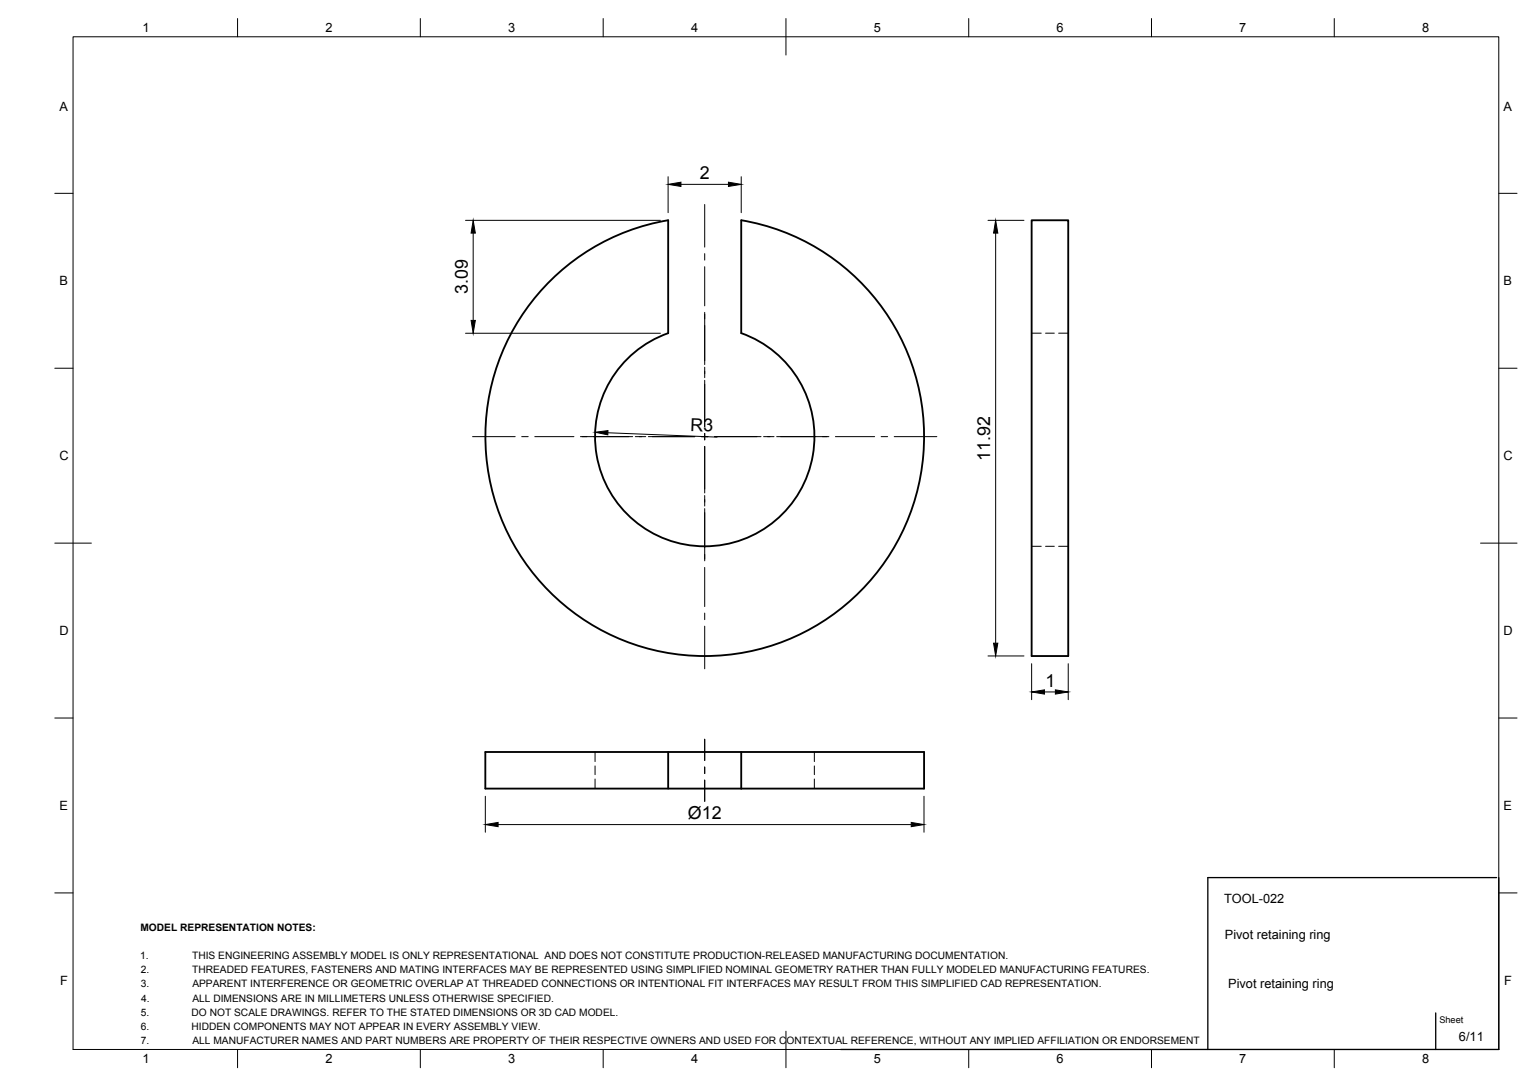
ISO-10303-21;
HEADER;
/* Generated by software containing ST-Developer
 * from STEP Tools, Inc. (www.steptools.com) 
 */

FILE_DESCRIPTION(
/* description */ (''),
/* implementation_level */ '2;1');

FILE_NAME(
/* name */ 'Pivot retaining ring.step',
/* time_stamp */ '2026-11-10T08:27:36-08:00',
/* author */ (''),
/* organization */ (''),
/* preprocessor_version */ 'ST-DEVELOPER v20.2',
/* originating_system */ 'Autodesk Translation Framework v15.17.0.0',
/* authorisation */ '');

FILE_SCHEMA (('AUTOMOTIVE_DESIGN { 1 0 10303 214 3 1 1 }'));
ENDSEC;

DATA;
#10=MECHANICAL_DESIGN_GEOMETRIC_PRESENTATION_REPRESENTATION('',(#569),#19090);
#549=SHAPE_REPRESENTATION_RELATIONSHIP('SRR','None',#19139,#559);
#559=ADVANCED_BREP_SHAPE_REPRESENTATION('',(#579),#19082);
#569=STYLED_ITEM('',(#19202),#579);
#579=MANIFOLD_SOLID_BREP('Body1',#6823);
#695=PLANE('',#7030);
#696=PLANE('',#7031);
#697=PLANE('',#7032);
#698=PLANE('',#7039);
#869=FACE_OUTER_BOUND('',#1272,.T.);
#870=FACE_OUTER_BOUND('',#1273,.T.);
#871=FACE_OUTER_BOUND('',#1274,.T.);
#872=FACE_OUTER_BOUND('',#1275,.T.);
#873=FACE_OUTER_BOUND('',#1276,.T.);
#874=FACE_OUTER_BOUND('',#1277,.T.);
#1272=EDGE_LOOP('',(#4609,#4610,#4611,#4612));
#1273=EDGE_LOOP('',(#4613,#4614,#4615,#4616));
#1274=EDGE_LOOP('',(#4617,#4618,#4619,#4620));
#1275=EDGE_LOOP('',(#4621,#4622,#4623,#4624));
#1276=EDGE_LOOP('',(#4625,#4626,#4627,#4628));
#1277=EDGE_LOOP('',(#4629,#4630,#4631,#4632));
#1765=LINE('',#9169,#2214);
#1766=LINE('',#9171,#2215);
#1767=LINE('',#9173,#2216);
#1768=LINE('',#9174,#2217);
#1769=LINE('',#9178,#2218);
#1770=LINE('',#9180,#2219);
#1771=LINE('',#9182,#2220);
#1772=LINE('',#9183,#2221);
#2214=VECTOR('',#7726,1.);
#2215=VECTOR('',#7727,1.);
#2216=VECTOR('',#7728,1.);
#2217=VECTOR('',#7729,1.);
#2218=VECTOR('',#7732,1.);
#2219=VECTOR('',#7733,1.);
#2220=VECTOR('',#7734,1.);
#2221=VECTOR('',#7735,1.);
#2582=CIRCLE('',#7033,0.6);
#2583=CIRCLE('',#7034,0.3);
#2584=CIRCLE('',#7036,0.3);
#2585=CIRCLE('',#7038,0.6);
#2804=VERTEX_POINT('',#9167);
#2805=VERTEX_POINT('',#9168);
#2806=VERTEX_POINT('',#9170);
#2807=VERTEX_POINT('',#9172);
#2808=VERTEX_POINT('',#9176);
#2809=VERTEX_POINT('',#9177);
#2810=VERTEX_POINT('',#9179);
#2811=VERTEX_POINT('',#9181);
#3489=EDGE_CURVE('',#2804,#2805,#1765,.T.);
#3490=EDGE_CURVE('',#2806,#2804,#1766,.T.);
#3491=EDGE_CURVE('',#2807,#2806,#1767,.T.);
#3492=EDGE_CURVE('',#2805,#2807,#1768,.T.);
#3493=EDGE_CURVE('',#2808,#2809,#1769,.T.);
#3494=EDGE_CURVE('',#2810,#2808,#1770,.T.);
#3495=EDGE_CURVE('',#2811,#2810,#1771,.T.);
#3496=EDGE_CURVE('',#2809,#2811,#1772,.T.);
#3497=EDGE_CURVE('',#2806,#2811,#2582,.T.);
#3498=EDGE_CURVE('',#2809,#2804,#2583,.T.);
#3499=EDGE_CURVE('',#2808,#2805,#2584,.T.);
#3500=EDGE_CURVE('',#2807,#2810,#2585,.T.);
#4609=ORIENTED_EDGE('',*,*,#3489,.F.);
#4610=ORIENTED_EDGE('',*,*,#3490,.F.);
#4611=ORIENTED_EDGE('',*,*,#3491,.F.);
#4612=ORIENTED_EDGE('',*,*,#3492,.F.);
#4613=ORIENTED_EDGE('',*,*,#3493,.F.);
#4614=ORIENTED_EDGE('',*,*,#3494,.F.);
#4615=ORIENTED_EDGE('',*,*,#3495,.F.);
#4616=ORIENTED_EDGE('',*,*,#3496,.F.);
#4617=ORIENTED_EDGE('',*,*,#3496,.T.);
#4618=ORIENTED_EDGE('',*,*,#3497,.F.);
#4619=ORIENTED_EDGE('',*,*,#3490,.T.);
#4620=ORIENTED_EDGE('',*,*,#3498,.F.);
#4621=ORIENTED_EDGE('',*,*,#3493,.T.);
#4622=ORIENTED_EDGE('',*,*,#3498,.T.);
#4623=ORIENTED_EDGE('',*,*,#3489,.T.);
#4624=ORIENTED_EDGE('',*,*,#3499,.F.);
#4625=ORIENTED_EDGE('',*,*,#3495,.T.);
#4626=ORIENTED_EDGE('',*,*,#3500,.F.);
#4627=ORIENTED_EDGE('',*,*,#3491,.T.);
#4628=ORIENTED_EDGE('',*,*,#3497,.T.);
#4629=ORIENTED_EDGE('',*,*,#3494,.T.);
#4630=ORIENTED_EDGE('',*,*,#3499,.T.);
#4631=ORIENTED_EDGE('',*,*,#3492,.T.);
#4632=ORIENTED_EDGE('',*,*,#3500,.T.);
#6315=CYLINDRICAL_SURFACE('',#7035,0.3);
#6316=CYLINDRICAL_SURFACE('',#7037,0.6);
#6488=ADVANCED_FACE('',(#869),#695,.F.);
#6489=ADVANCED_FACE('',(#870),#696,.F.);
#6490=ADVANCED_FACE('',(#871),#697,.F.);
#6491=ADVANCED_FACE('',(#872),#6315,.F.);
#6492=ADVANCED_FACE('',(#873),#6316,.T.);
#6493=ADVANCED_FACE('',(#874),#698,.T.);
#6823=CLOSED_SHELL('',(#6488,#6489,#6490,#6491,#6492,#6493));
#7029=AXIS2_PLACEMENT_3D('',#9165,#7722,#7723);
#7030=AXIS2_PLACEMENT_3D('',#9166,#7724,#7725);
#7031=AXIS2_PLACEMENT_3D('',#9175,#7730,#7731);
#7032=AXIS2_PLACEMENT_3D('',#9184,#7736,#7737);
#7033=AXIS2_PLACEMENT_3D('',#9185,#7738,#7739);
#7034=AXIS2_PLACEMENT_3D('',#9186,#7740,#7741);
#7035=AXIS2_PLACEMENT_3D('',#9187,#7742,#7743);
#7036=AXIS2_PLACEMENT_3D('',#9188,#7744,#7745);
#7037=AXIS2_PLACEMENT_3D('',#9189,#7746,#7747);
#7038=AXIS2_PLACEMENT_3D('',#9190,#7748,#7749);
#7039=AXIS2_PLACEMENT_3D('',#9191,#7750,#7751);
#7722=DIRECTION('axis',(0.,0.,1.));
#7723=DIRECTION('refdir',(1.,0.,0.));
#7724=DIRECTION('center_axis',(-1.,0.,0.));
#7725=DIRECTION('ref_axis',(0.,1.,0.));
#7726=DIRECTION('',(0.,0.,1.));
#7727=DIRECTION('',(0.,-1.,0.));
#7728=DIRECTION('',(0.,0.,-1.));
#7729=DIRECTION('',(0.,1.,0.));
#7730=DIRECTION('center_axis',(1.,0.,0.));
#7731=DIRECTION('ref_axis',(0.,-1.,0.));
#7732=DIRECTION('',(0.,0.,-1.));
#7733=DIRECTION('',(0.,-1.,0.));
#7734=DIRECTION('',(0.,0.,1.));
#7735=DIRECTION('',(0.,1.,0.));
#7736=DIRECTION('center_axis',(0.,0.,1.));
#7737=DIRECTION('ref_axis',(1.,0.,0.));
#7738=DIRECTION('center_axis',(0.,0.,1.));
#7739=DIRECTION('ref_axis',(1.,0.,0.));
#7740=DIRECTION('center_axis',(0.,0.,-1.));
#7741=DIRECTION('ref_axis',(1.,0.,0.));
#7742=DIRECTION('center_axis',(0.,0.,1.));
#7743=DIRECTION('ref_axis',(6.12323399573677E-17,-1.,0.));
#7744=DIRECTION('center_axis',(0.,0.,-1.));
#7745=DIRECTION('ref_axis',(1.,0.,0.));
#7746=DIRECTION('center_axis',(0.,0.,1.));
#7747=DIRECTION('ref_axis',(6.12323399573677E-17,-1.,0.));
#7748=DIRECTION('center_axis',(0.,0.,1.));
#7749=DIRECTION('ref_axis',(1.,0.,0.));
#7750=DIRECTION('center_axis',(0.,0.,1.));
#7751=DIRECTION('ref_axis',(1.,0.,0.));
#9165=CARTESIAN_POINT('',(0.,0.,0.));
#9166=CARTESIAN_POINT('Origin',(-0.1,0.,0.1));
#9167=CARTESIAN_POINT('',(-0.1,0.282842712474619,0.));
#9168=CARTESIAN_POINT('',(-0.1,0.282842712474619,0.1));
#9169=CARTESIAN_POINT('',(-0.1,0.282842712474619,0.));
#9170=CARTESIAN_POINT('',(-0.1,0.591607978309962,0.));
#9171=CARTESIAN_POINT('',(-0.1,0.,0.));
#9172=CARTESIAN_POINT('',(-0.1,0.591607978309962,0.1));
#9173=CARTESIAN_POINT('',(-0.1,0.591607978309962,0.));
#9174=CARTESIAN_POINT('',(-0.1,0.,0.1));
#9175=CARTESIAN_POINT('Origin',(0.1,1.2,0.1));
#9176=CARTESIAN_POINT('',(0.1,0.282842712474619,0.1));
#9177=CARTESIAN_POINT('',(0.1,0.282842712474619,0.));
#9178=CARTESIAN_POINT('',(0.1,0.282842712474619,0.));
#9179=CARTESIAN_POINT('',(0.1,0.591607978309962,0.1));
#9180=CARTESIAN_POINT('',(0.1,0.6,0.1));
#9181=CARTESIAN_POINT('',(0.1,0.591607978309962,0.));
#9182=CARTESIAN_POINT('',(0.1,0.591607978309962,0.));
#9183=CARTESIAN_POINT('',(0.1,0.6,0.));
#9184=CARTESIAN_POINT('Origin',(0.,0.,0.));
#9185=CARTESIAN_POINT('Origin',(0.,0.,0.));
#9186=CARTESIAN_POINT('Origin',(0.,0.,0.));
#9187=CARTESIAN_POINT('Origin',(0.,0.,0.));
#9188=CARTESIAN_POINT('Origin',(0.,0.,0.1));
#9189=CARTESIAN_POINT('Origin',(0.,0.,0.));
#9190=CARTESIAN_POINT('Origin',(0.,0.,0.1));
#9191=CARTESIAN_POINT('Origin',(0.,0.,0.1));
#19069=UNCERTAINTY_MEASURE_WITH_UNIT(LENGTH_MEASURE(0.001),#19091,
'DISTANCE_ACCURACY_VALUE',
'Maximum model space distance between geometric entities at asserted c
onnectivities');
#19077=UNCERTAINTY_MEASURE_WITH_UNIT(LENGTH_MEASURE(0.001),#19091,
'DISTANCE_ACCURACY_VALUE',
'Maximum model space distance between geometric entities at asserted c
onnectivities');
#19082=(
GEOMETRIC_REPRESENTATION_CONTEXT(3)
GLOBAL_UNCERTAINTY_ASSIGNED_CONTEXT((#19069))
GLOBAL_UNIT_ASSIGNED_CONTEXT((#19091,#19093,#19094))
REPRESENTATION_CONTEXT('','3D')
);
#19090=(
GEOMETRIC_REPRESENTATION_CONTEXT(3)
GLOBAL_UNCERTAINTY_ASSIGNED_CONTEXT((#19077))
GLOBAL_UNIT_ASSIGNED_CONTEXT((#19091,#19093,#19094))
REPRESENTATION_CONTEXT('','3D')
);
#19091=(
LENGTH_UNIT()
NAMED_UNIT(*)
SI_UNIT(.CENTI.,.METRE.)
);
#19093=(
NAMED_UNIT(*)
PLANE_ANGLE_UNIT()
SI_UNIT($,.RADIAN.)
);
#19094=(
NAMED_UNIT(*)
SI_UNIT($,.STERADIAN.)
SOLID_ANGLE_UNIT()
);
#19099=SHAPE_DEFINITION_REPRESENTATION(#19111,#19139);
#19111=PRODUCT_DEFINITION_SHAPE('',$,#19152);
#19139=SHAPE_REPRESENTATION('',(#7029),#19082);
#19147=PRODUCT_DEFINITION_CONTEXT('part definition',#19185,'design');
#19152=PRODUCT_DEFINITION('Pivot retaining ring','Pivot retaining ring',
#19164,#19147);
#19164=PRODUCT_DEFINITION_FORMATION('',$,#19191);
#19185=APPLICATION_CONTEXT(
'Core Data for Automotive Mechanical Design Process');
#19186=PRODUCT_CONTEXT('part definition',#19185,'mechanical');
#19191=PRODUCT('Pivot retaining ring','Pivot retaining ring',$,(#19186));
#19202=PRESENTATION_STYLE_ASSIGNMENT((#19210));
#19210=SURFACE_STYLE_USAGE(.BOTH.,#19218);
#19218=SURFACE_SIDE_STYLE('',(#19226));
#19226=SURFACE_STYLE_FILL_AREA(#19234);
#19234=FILL_AREA_STYLE('Dark gray',(#19242));
#19242=FILL_AREA_STYLE_COLOUR('Dark gray',#19250);
#19250=COLOUR_RGB('Dark gray',0.250980392156863,0.282352941176471,0.32156862745098);
ENDSEC;
END-ISO-10303-21;
